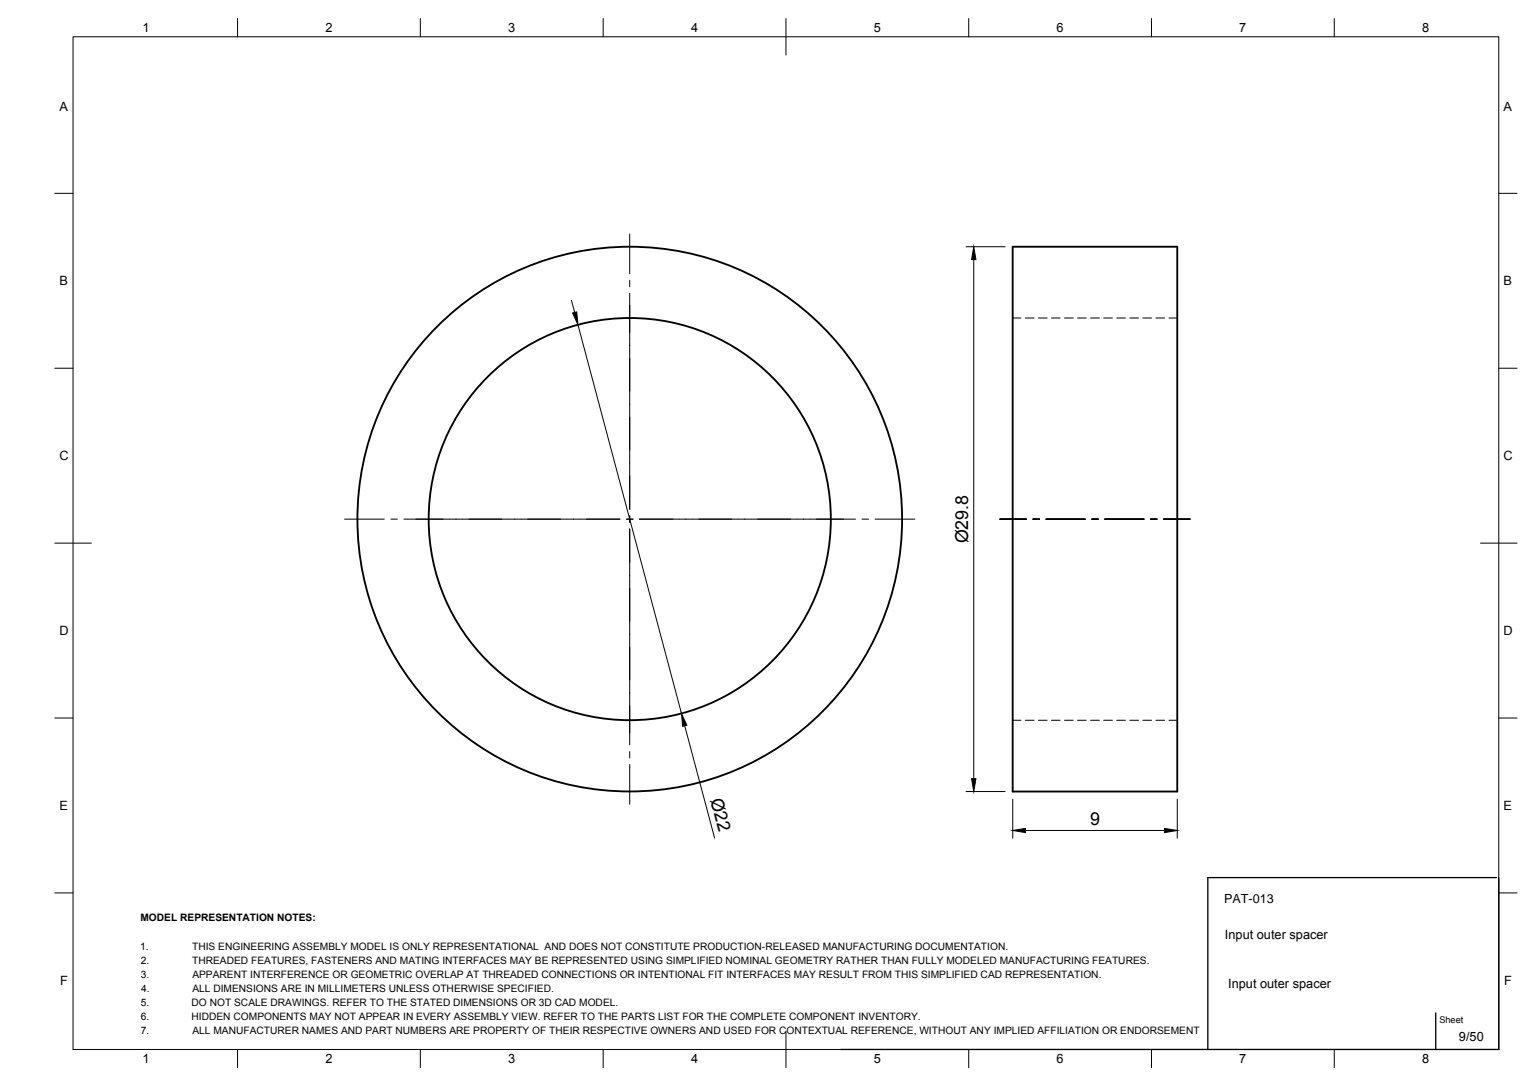
ISO-10303-21;
HEADER;
/* Generated by software containing ST-Developer
 * from STEP Tools, Inc. (www.steptools.com) 
 */

FILE_DESCRIPTION(
/* description */ ('Belt-driven linear axis on 2020 extrusion'),
/* implementation_level */ '2;1');

FILE_NAME(
/* name */ 'Input outer spacer.step',
/* time_stamp */ '2026-10-28T03:26:09-07:00',
/* author */ (''),
/* organization */ (''),
/* preprocessor_version */ 'ST-DEVELOPER v20.2',
/* originating_system */ 'Autodesk Translation Framework v15.17.0.0',
/* authorisation */ '');

FILE_SCHEMA (('AUTOMOTIVE_DESIGN { 1 0 10303 214 3 1 1 }'));
ENDSEC;

DATA;
#10=MECHANICAL_DESIGN_GEOMETRIC_PRESENTATION_REPRESENTATION('',(#616),#20096);
#522=SHAPE_REPRESENTATION_RELATIONSHIP('SRR','None',#20318,#568);
#568=ADVANCED_BREP_SHAPE_REPRESENTATION('',(#672),#20049);
#616=STYLED_ITEM('',(#20643),#672);
#672=MANIFOLD_SOLID_BREP('Body1',#10929);
#760=FACE_BOUND('',#2002,.T.);
#761=FACE_BOUND('',#2004,.T.);
#945=PLANE('',#11646);
#946=PLANE('',#11647);
#1335=FACE_OUTER_BOUND('',#1999,.T.);
#1336=FACE_OUTER_BOUND('',#2000,.T.);
#1337=FACE_OUTER_BOUND('',#2001,.T.);
#1338=FACE_OUTER_BOUND('',#2003,.T.);
#1999=EDGE_LOOP('',(#7595,#7596,#7597,#7598));
#2000=EDGE_LOOP('',(#7599,#7600,#7601,#7602));
#2001=EDGE_LOOP('',(#7603));
#2002=EDGE_LOOP('',(#7604));
#2003=EDGE_LOOP('',(#7605));
#2004=EDGE_LOOP('',(#7606));
#2778=LINE('',#16613,#3635);
#2779=LINE('',#16619,#3636);
#3635=VECTOR('',#13202,1.1);
#3636=VECTOR('',#13209,1.49);
#4437=CIRCLE('',#11641,1.1);
#4438=CIRCLE('',#11642,1.1);
#4439=CIRCLE('',#11644,1.49);
#4440=CIRCLE('',#11645,1.49);
#5006=VERTEX_POINT('',#16610);
#5007=VERTEX_POINT('',#16612);
#5008=VERTEX_POINT('',#16616);
#5009=VERTEX_POINT('',#16618);
#6012=EDGE_CURVE('',#5006,#5006,#4437,.T.);
#6013=EDGE_CURVE('',#5006,#5007,#2778,.T.);
#6014=EDGE_CURVE('',#5007,#5007,#4438,.T.);
#6015=EDGE_CURVE('',#5008,#5008,#4439,.T.);
#6016=EDGE_CURVE('',#5008,#5009,#2779,.T.);
#6017=EDGE_CURVE('',#5009,#5009,#4440,.T.);
#7595=ORIENTED_EDGE('',*,*,#6012,.F.);
#7596=ORIENTED_EDGE('',*,*,#6013,.T.);
#7597=ORIENTED_EDGE('',*,*,#6014,.T.);
#7598=ORIENTED_EDGE('',*,*,#6013,.F.);
#7599=ORIENTED_EDGE('',*,*,#6015,.F.);
#7600=ORIENTED_EDGE('',*,*,#6016,.T.);
#7601=ORIENTED_EDGE('',*,*,#6017,.T.);
#7602=ORIENTED_EDGE('',*,*,#6016,.F.);
#7603=ORIENTED_EDGE('',*,*,#6015,.T.);
#7604=ORIENTED_EDGE('',*,*,#6012,.T.);
#7605=ORIENTED_EDGE('',*,*,#6017,.F.);
#7606=ORIENTED_EDGE('',*,*,#6014,.F.);
#10106=CYLINDRICAL_SURFACE('',#11640,1.1);
#10107=CYLINDRICAL_SURFACE('',#11643,1.49);
#10386=ADVANCED_FACE('',(#1335),#10106,.F.);
#10387=ADVANCED_FACE('',(#1336),#10107,.T.);
#10388=ADVANCED_FACE('',(#1337,#760),#945,.T.);
#10389=ADVANCED_FACE('',(#1338,#761),#946,.F.);
#10929=CLOSED_SHELL('',(#10386,#10387,#10388,#10389));
#11639=AXIS2_PLACEMENT_3D('',#16608,#13196,#13197);
#11640=AXIS2_PLACEMENT_3D('',#16609,#13198,#13199);
#11641=AXIS2_PLACEMENT_3D('',#16611,#13200,#13201);
#11642=AXIS2_PLACEMENT_3D('',#16614,#13203,#13204);
#11643=AXIS2_PLACEMENT_3D('',#16615,#13205,#13206);
#11644=AXIS2_PLACEMENT_3D('',#16617,#13207,#13208);
#11645=AXIS2_PLACEMENT_3D('',#16620,#13210,#13211);
#11646=AXIS2_PLACEMENT_3D('',#16621,#13212,#13213);
#11647=AXIS2_PLACEMENT_3D('',#16622,#13214,#13215);
#13196=DIRECTION('axis',(0.,0.,1.));
#13197=DIRECTION('refdir',(1.,0.,0.));
#13198=DIRECTION('center_axis',(0.,1.,0.));
#13199=DIRECTION('ref_axis',(1.,0.,0.));
#13200=DIRECTION('center_axis',(0.,-1.,0.));
#13201=DIRECTION('ref_axis',(1.,0.,0.));
#13202=DIRECTION('',(0.,-1.,0.));
#13203=DIRECTION('center_axis',(0.,-1.,0.));
#13204=DIRECTION('ref_axis',(1.,0.,0.));
#13205=DIRECTION('center_axis',(0.,1.,0.));
#13206=DIRECTION('ref_axis',(1.,0.,0.));
#13207=DIRECTION('center_axis',(0.,1.,0.));
#13208=DIRECTION('ref_axis',(1.,0.,0.));
#13209=DIRECTION('',(0.,-1.,0.));
#13210=DIRECTION('center_axis',(0.,1.,0.));
#13211=DIRECTION('ref_axis',(1.,0.,0.));
#13212=DIRECTION('center_axis',(0.,1.,0.));
#13213=DIRECTION('ref_axis',(1.,0.,0.));
#13214=DIRECTION('center_axis',(0.,1.,0.));
#13215=DIRECTION('ref_axis',(1.,0.,0.));
#16608=CARTESIAN_POINT('',(0.,0.,0.));
#16609=CARTESIAN_POINT('Origin',(0.,-0.45,7.));
#16610=CARTESIAN_POINT('',(-1.1,0.45,7.));
#16611=CARTESIAN_POINT('Origin',(0.,0.45,7.));
#16612=CARTESIAN_POINT('',(-1.1,-0.45,7.));
#16613=CARTESIAN_POINT('',(-1.1,-0.45,7.));
#16614=CARTESIAN_POINT('Origin',(0.,-0.45,7.));
#16615=CARTESIAN_POINT('Origin',(0.,-0.45,7.));
#16616=CARTESIAN_POINT('',(-1.49,0.45,7.));
#16617=CARTESIAN_POINT('Origin',(0.,0.45,7.));
#16618=CARTESIAN_POINT('',(-1.49,-0.45,7.));
#16619=CARTESIAN_POINT('',(-1.49,-0.45,7.));
#16620=CARTESIAN_POINT('Origin',(0.,-0.45,7.));
#16621=CARTESIAN_POINT('Origin',(0.,0.45,7.));
#16622=CARTESIAN_POINT('Origin',(0.,-0.45,7.));
#19995=UNCERTAINTY_MEASURE_WITH_UNIT(LENGTH_MEASURE(0.001),#20097,
'DISTANCE_ACCURACY_VALUE',
'Maximum model space distance between geometric entities at asserted c
onnectivities');
#20042=UNCERTAINTY_MEASURE_WITH_UNIT(LENGTH_MEASURE(0.001),#20097,
'DISTANCE_ACCURACY_VALUE',
'Maximum model space distance between geometric entities at asserted c
onnectivities');
#20049=(
GEOMETRIC_REPRESENTATION_CONTEXT(3)
GLOBAL_UNCERTAINTY_ASSIGNED_CONTEXT((#19995))
GLOBAL_UNIT_ASSIGNED_CONTEXT((#20097,#20099,#20100))
REPRESENTATION_CONTEXT('','3D')
);
#20096=(
GEOMETRIC_REPRESENTATION_CONTEXT(3)
GLOBAL_UNCERTAINTY_ASSIGNED_CONTEXT((#20042))
GLOBAL_UNIT_ASSIGNED_CONTEXT((#20097,#20099,#20100))
REPRESENTATION_CONTEXT('','3D')
);
#20097=(
LENGTH_UNIT()
NAMED_UNIT(*)
SI_UNIT(.CENTI.,.METRE.)
);
#20099=(
NAMED_UNIT(*)
PLANE_ANGLE_UNIT()
SI_UNIT($,.RADIAN.)
);
#20100=(
NAMED_UNIT(*)
SI_UNIT($,.STERADIAN.)
SOLID_ANGLE_UNIT()
);
#20107=SHAPE_DEFINITION_REPRESENTATION(#20160,#20318);
#20160=PRODUCT_DEFINITION_SHAPE('',$,#20372);
#20318=SHAPE_REPRESENTATION('',(#11639),#20049);
#20365=PRODUCT_DEFINITION_CONTEXT('part definition',#20526,'design');
#20372=PRODUCT_DEFINITION('Input outer spacer','Input outer spacer',#20425,
#20365);
#20425=PRODUCT_DEFINITION_FORMATION('',$,#20534);
#20526=APPLICATION_CONTEXT(
'Core Data for Automotive Mechanical Design Process');
#20527=PRODUCT_CONTEXT('part definition',#20526,'mechanical');
#20534=PRODUCT('Input outer spacer','Input outer spacer',
'Input outer spacer',(#20527));
#20637=COLOUR_RGB('Sky Blue',0.24,0.69,0.87);
#20638=FILL_AREA_STYLE_COLOUR('',#20637);
#20639=FILL_AREA_STYLE('',(#20638));
#20640=SURFACE_STYLE_FILL_AREA(#20639);
#20641=SURFACE_SIDE_STYLE('',(#20640));
#20642=SURFACE_STYLE_USAGE(.BOTH.,#20641);
#20643=PRESENTATION_STYLE_ASSIGNMENT((#20642));
ENDSEC;
END-ISO-10303-21;
